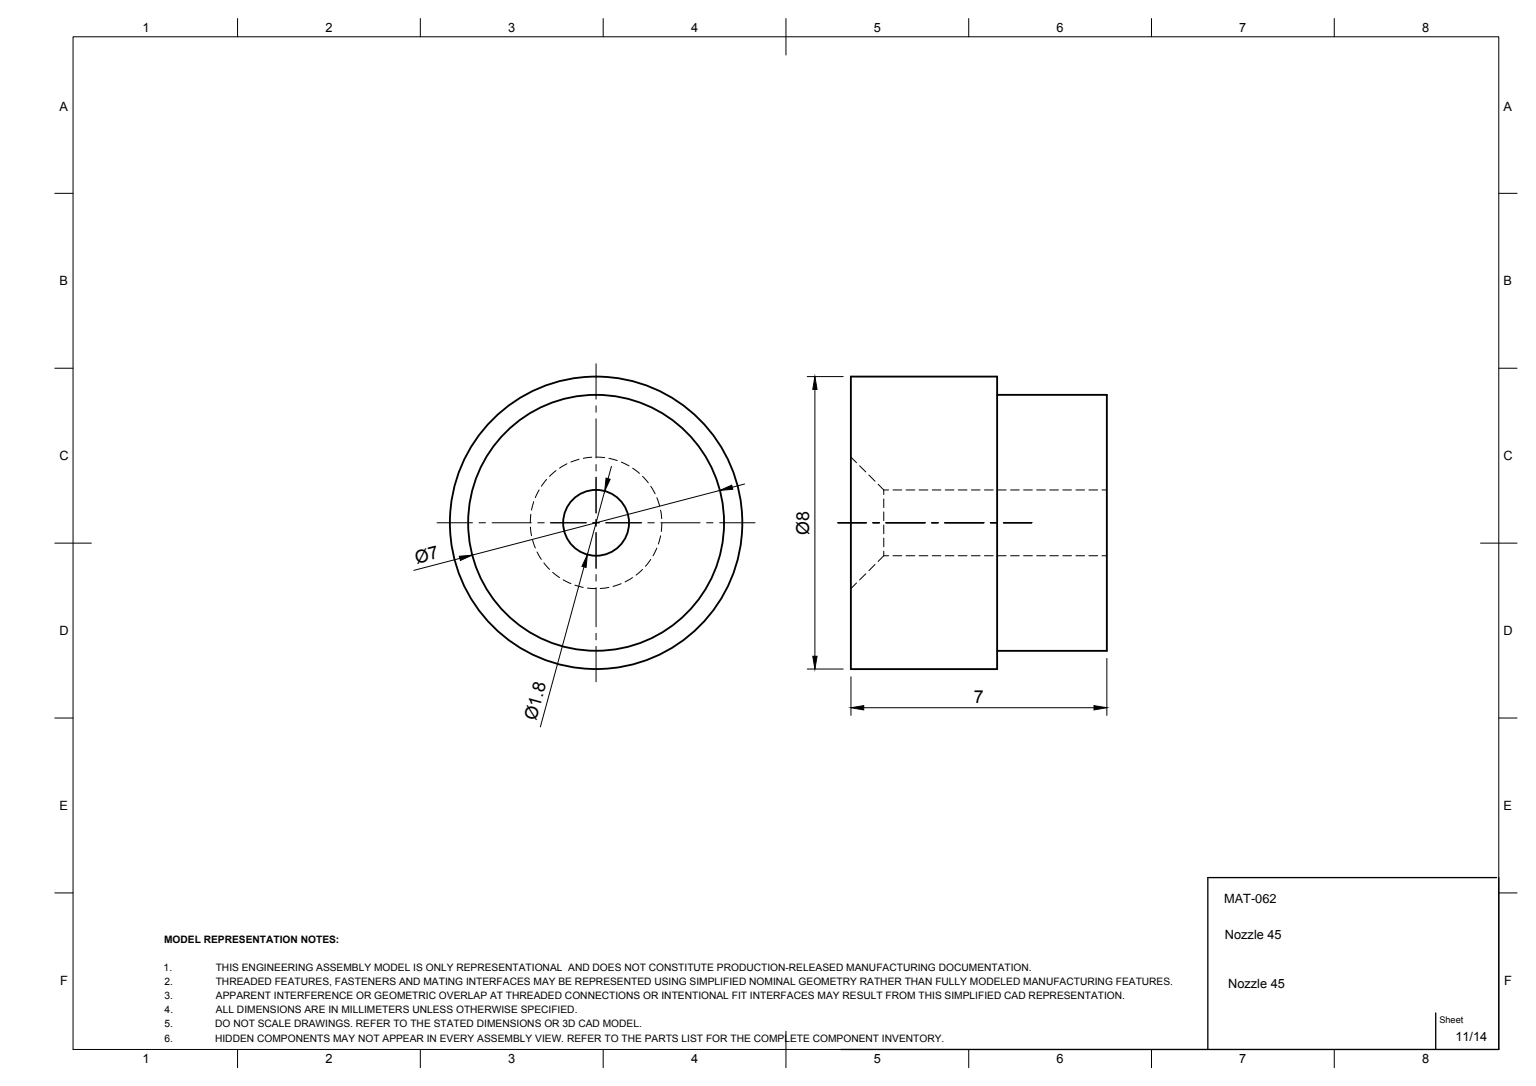
ISO-10303-21;
HEADER;
/* Generated by software containing ST-Developer
 * from STEP Tools, Inc. (www.steptools.com) 
 */

FILE_DESCRIPTION(
/* description */ (''),
/* implementation_level */ '2;1');

FILE_NAME(
/* name */ 'Nozzle 45.step',
/* time_stamp */ '2026-10-24T10:18:25-07:00',
/* author */ (''),
/* organization */ (''),
/* preprocessor_version */ 'ST-DEVELOPER v20.2',
/* originating_system */ 'Autodesk Translation Framework v15.15.0.0',
/* authorisation */ '');

FILE_SCHEMA (('AUTOMOTIVE_DESIGN { 1 0 10303 214 3 1 1 }'));
ENDSEC;

DATA;
#10=MECHANICAL_DESIGN_GEOMETRIC_PRESENTATION_REPRESENTATION('',(#261),#14125);
#195=CONICAL_SURFACE('',#6635,1.8,0.785398163397447);
#232=SHAPE_REPRESENTATION_RELATIONSHIP('SRR','None',#14206,#242);
#242=ADVANCED_BREP_SHAPE_REPRESENTATION('',(#274),#14120);
#261=STYLED_ITEM('',(#14263),#274);
#274=MANIFOLD_SOLID_BREP('Nozzle 45',#6142);
#557=CYLINDRICAL_SURFACE('',#6625,4.00000000000001);
#558=CYLINDRICAL_SURFACE('',#6632,0.899999999999993);
#559=CYLINDRICAL_SURFACE('',#6638,3.50000000000001);
#678=FACE_BOUND('',#1352,.T.);
#679=FACE_BOUND('',#1354,.T.);
#680=FACE_BOUND('',#1358,.T.);
#946=FACE_OUTER_BOUND('',#1350,.T.);
#947=FACE_OUTER_BOUND('',#1351,.T.);
#948=FACE_OUTER_BOUND('',#1353,.T.);
#949=FACE_OUTER_BOUND('',#1355,.T.);
#950=FACE_OUTER_BOUND('',#1356,.T.);
#951=FACE_OUTER_BOUND('',#1357,.T.);
#952=FACE_OUTER_BOUND('',#1359,.T.);
#1350=EDGE_LOOP('',(#5003,#5004,#5005,#5006));
#1351=EDGE_LOOP('',(#5007));
#1352=EDGE_LOOP('',(#5008));
#1353=EDGE_LOOP('',(#5009));
#1354=EDGE_LOOP('',(#5010));
#1355=EDGE_LOOP('',(#5011,#5012,#5013,#5014));
#1356=EDGE_LOOP('',(#5015,#5016,#5017,#5018));
#1357=EDGE_LOOP('',(#5019));
#1358=EDGE_LOOP('',(#5020));
#1359=EDGE_LOOP('',(#5021,#5022,#5023,#5024));
#1706=CIRCLE('',#6626,4.00000000000001);
#1707=CIRCLE('',#6627,4.00000000000001);
#1708=CIRCLE('',#6629,3.50000000000001);
#1709=CIRCLE('',#6631,1.8);
#1710=CIRCLE('',#6633,0.899999999999997);
#1711=CIRCLE('',#6634,0.899999999999995);
#1712=CIRCLE('',#6637,3.50000000000001);
#2042=LINE('',#12244,#2430);
#2043=LINE('',#12256,#2431);
#2044=LINE('',#12259,#2432);
#2045=LINE('',#12264,#2433);
#2430=VECTOR('',#7884,4.00000000000001);
#2431=VECTOR('',#7899,0.899999999999993);
#2432=VECTOR('',#7904,1.8);
#2433=VECTOR('',#7911,3.50000000000002);
#2923=VERTEX_POINT('',#12241);
#2924=VERTEX_POINT('',#12243);
#2925=VERTEX_POINT('',#12247);
#2926=VERTEX_POINT('',#12250);
#2927=VERTEX_POINT('',#12253);
#2928=VERTEX_POINT('',#12255);
#2929=VERTEX_POINT('',#12261);
#3649=EDGE_CURVE('',#2923,#2923,#1706,.T.);
#3650=EDGE_CURVE('',#2923,#2924,#2042,.T.);
#3651=EDGE_CURVE('',#2924,#2924,#1707,.T.);
#3652=EDGE_CURVE('',#2925,#2925,#1708,.T.);
#3653=EDGE_CURVE('',#2926,#2926,#1709,.T.);
#3654=EDGE_CURVE('',#2927,#2927,#1710,.T.);
#3655=EDGE_CURVE('',#2927,#2928,#2043,.T.);
#3656=EDGE_CURVE('',#2928,#2928,#1711,.T.);
#3657=EDGE_CURVE('',#2928,#2926,#2044,.T.);
#3658=EDGE_CURVE('',#2929,#2929,#1712,.T.);
#3659=EDGE_CURVE('',#2925,#2929,#2045,.T.);
#5003=ORIENTED_EDGE('',*,*,#3649,.T.);
#5004=ORIENTED_EDGE('',*,*,#3650,.T.);
#5005=ORIENTED_EDGE('',*,*,#3651,.F.);
#5006=ORIENTED_EDGE('',*,*,#3650,.F.);
#5007=ORIENTED_EDGE('',*,*,#3651,.T.);
#5008=ORIENTED_EDGE('',*,*,#3652,.F.);
#5009=ORIENTED_EDGE('',*,*,#3649,.F.);
#5010=ORIENTED_EDGE('',*,*,#3653,.F.);
#5011=ORIENTED_EDGE('',*,*,#3654,.T.);
#5012=ORIENTED_EDGE('',*,*,#3655,.T.);
#5013=ORIENTED_EDGE('',*,*,#3656,.T.);
#5014=ORIENTED_EDGE('',*,*,#3655,.F.);
#5015=ORIENTED_EDGE('',*,*,#3656,.F.);
#5016=ORIENTED_EDGE('',*,*,#3657,.T.);
#5017=ORIENTED_EDGE('',*,*,#3653,.T.);
#5018=ORIENTED_EDGE('',*,*,#3657,.F.);
#5019=ORIENTED_EDGE('',*,*,#3658,.T.);
#5020=ORIENTED_EDGE('',*,*,#3654,.F.);
#5021=ORIENTED_EDGE('',*,*,#3652,.T.);
#5022=ORIENTED_EDGE('',*,*,#3659,.T.);
#5023=ORIENTED_EDGE('',*,*,#3658,.F.);
#5024=ORIENTED_EDGE('',*,*,#3659,.F.);
#5719=PLANE('',#6628);
#5720=PLANE('',#6630);
#5721=PLANE('',#6636);
#5995=ADVANCED_FACE('',(#946),#557,.T.);
#5996=ADVANCED_FACE('',(#947,#678),#5719,.T.);
#5997=ADVANCED_FACE('',(#948,#679),#5720,.F.);
#5998=ADVANCED_FACE('',(#949),#558,.F.);
#5999=ADVANCED_FACE('',(#950),#195,.F.);
#6000=ADVANCED_FACE('',(#951,#680),#5721,.T.);
#6001=ADVANCED_FACE('',(#952),#559,.T.);
#6142=CLOSED_SHELL('',(#5995,#5996,#5997,#5998,#5999,#6000,#6001));
#6624=AXIS2_PLACEMENT_3D('',#12239,#7878,#7879);
#6625=AXIS2_PLACEMENT_3D('',#12240,#7880,#7881);
#6626=AXIS2_PLACEMENT_3D('',#12242,#7882,#7883);
#6627=AXIS2_PLACEMENT_3D('',#12245,#7885,#7886);
#6628=AXIS2_PLACEMENT_3D('',#12246,#7887,#7888);
#6629=AXIS2_PLACEMENT_3D('',#12248,#7889,#7890);
#6630=AXIS2_PLACEMENT_3D('',#12249,#7891,#7892);
#6631=AXIS2_PLACEMENT_3D('',#12251,#7893,#7894);
#6632=AXIS2_PLACEMENT_3D('',#12252,#7895,#7896);
#6633=AXIS2_PLACEMENT_3D('',#12254,#7897,#7898);
#6634=AXIS2_PLACEMENT_3D('',#12257,#7900,#7901);
#6635=AXIS2_PLACEMENT_3D('',#12258,#7902,#7903);
#6636=AXIS2_PLACEMENT_3D('',#12260,#7905,#7906);
#6637=AXIS2_PLACEMENT_3D('',#12262,#7907,#7908);
#6638=AXIS2_PLACEMENT_3D('',#12263,#7909,#7910);
#7878=DIRECTION('axis',(0.,0.,1.));
#7879=DIRECTION('refdir',(1.,0.,0.));
#7880=DIRECTION('center_axis',(-0.612372435695796,0.707106781186546,-0.353553390593275));
#7881=DIRECTION('ref_axis',(-0.755928946018453,-0.654653670707979,0.));
#7882=DIRECTION('center_axis',(0.612372435695796,-0.707106781186546,0.353553390593275));
#7883=DIRECTION('ref_axis',(0.755928946018453,0.654653670707979,0.));
#7884=DIRECTION('',(0.612372435695796,-0.707106781186546,0.353553390593275));
#7885=DIRECTION('center_axis',(0.612372435695796,-0.707106781186546,0.353553390593275));
#7886=DIRECTION('ref_axis',(0.755928946018453,0.654653670707979,0.));
#7887=DIRECTION('center_axis',(0.612372435695796,-0.707106781186546,0.353553390593275));
#7888=DIRECTION('ref_axis',(0.5,0.,-0.866025403784438));
#7889=DIRECTION('center_axis',(0.612372435695796,-0.707106781186546,0.353553390593275));
#7890=DIRECTION('ref_axis',(0.755928946018453,0.654653670707979,0.));
#7891=DIRECTION('center_axis',(0.612372435695796,-0.707106781186546,0.353553390593275));
#7892=DIRECTION('ref_axis',(0.5,0.,-0.866025403784438));
#7893=DIRECTION('center_axis',(-0.612372435695796,0.707106781186546,-0.353553390593275));
#7894=DIRECTION('ref_axis',(-0.755928946018453,-0.654653670707979,0.));
#7895=DIRECTION('center_axis',(-0.612372435695796,0.707106781186546,-0.353553390593275));
#7896=DIRECTION('ref_axis',(-0.755928946018453,-0.654653670707979,0.));
#7897=DIRECTION('center_axis',(0.612372435695796,-0.707106781186546,0.353553390593275));
#7898=DIRECTION('ref_axis',(0.755928946018453,0.654653670707979,0.));
#7899=DIRECTION('',(-0.612372435695796,0.707106781186546,-0.353553390593275));
#7900=DIRECTION('center_axis',(-0.612372435695796,0.707106781186546,-0.353553390593275));
#7901=DIRECTION('ref_axis',(-0.755928946018453,-0.654653670707979,0.));
#7902=DIRECTION('center_axis',(-0.612372435695796,0.707106781186546,-0.353553390593275));
#7903=DIRECTION('ref_axis',(-0.755928946018453,-0.654653670707979,0.));
#7904=DIRECTION('',(0.101509781932626,0.962910049886276,-0.250000000000001));
#7905=DIRECTION('center_axis',(0.612372435695796,-0.707106781186546,0.353553390593275));
#7906=DIRECTION('ref_axis',(0.5,0.,-0.866025403784438));
#7907=DIRECTION('center_axis',(0.612372435695796,-0.707106781186546,0.353553390593275));
#7908=DIRECTION('ref_axis',(0.755928946018453,0.654653670707979,0.));
#7909=DIRECTION('center_axis',(-0.612372435695796,0.707106781186546,-0.353553390593275));
#7910=DIRECTION('ref_axis',(-0.755928946018453,-0.654653670707979,0.));
#7911=DIRECTION('',(0.612372435695796,-0.707106781186546,0.353553390593275));
#12239=CARTESIAN_POINT('',(0.,0.,0.));
#12240=CARTESIAN_POINT('Origin',(-116.12807069331,130.343145750508,-79.0465728752519));
#12241=CARTESIAN_POINT('',(-115.553844652019,135.790187558086,-80.460786437625));
#12242=CARTESIAN_POINT('Origin',(-118.577560436093,133.171572875254,-80.460786437625));
#12243=CARTESIAN_POINT('',(-113.104354909236,132.96176043334,-79.0465728752519));
#12244=CARTESIAN_POINT('',(-113.104354909236,132.96176043334,-79.0465728752519));
#12245=CARTESIAN_POINT('Origin',(-116.12807069331,130.343145750508,-79.0465728752519));
#12246=CARTESIAN_POINT('Origin',(-116.12807069331,130.343145750508,-79.0465728752519));
#12247=CARTESIAN_POINT('',(-113.482319382245,132.634433597986,-79.0465728752519));
#12248=CARTESIAN_POINT('Origin',(-116.12807069331,130.343145750508,-79.0465728752519));
#12249=CARTESIAN_POINT('Origin',(-118.577560436093,133.171572875254,-80.460786437625));
#12250=CARTESIAN_POINT('',(-117.21688833326,134.349949482528,-80.460786437625));
#12251=CARTESIAN_POINT('Origin',(-118.577560436093,133.171572875254,-80.460786437625));
#12252=CARTESIAN_POINT('Origin',(-118.577560436093,133.171572875254,-80.460786437625));
#12253=CARTESIAN_POINT('',(-113.610617334806,128.811013710585,-77.9859127034721));
#12254=CARTESIAN_POINT('Origin',(-114.290953386223,128.221825406948,-77.9859127034721));
#12255=CARTESIAN_POINT('',(-117.34608919255,133.124365075823,-80.1425883860911));
#12256=CARTESIAN_POINT('',(-117.897224384677,133.760761178891,-80.460786437625));
#12257=CARTESIAN_POINT('Origin',(-118.026425243967,132.535176772186,-80.1425883860911));
#12258=CARTESIAN_POINT('Origin',(-118.577560436093,133.171572875254,-80.460786437625));
#12259=CARTESIAN_POINT('',(-117.21688833326,134.349949482528,-80.460786437625));
#12260=CARTESIAN_POINT('Origin',(-114.290953386223,128.221825406948,-77.9859127034721));
#12261=CARTESIAN_POINT('',(-111.645202075158,130.513113254426,-77.9859127034721));
#12262=CARTESIAN_POINT('Origin',(-114.290953386223,128.221825406948,-77.9859127034721));
#12263=CARTESIAN_POINT('Origin',(-114.290953386223,128.221825406948,-77.9859127034721));
#12264=CARTESIAN_POINT('',(-111.645202075158,130.513113254426,-77.9859127034721));
#14107=UNCERTAINTY_MEASURE_WITH_UNIT(LENGTH_MEASURE(0.01),#14126,
'DISTANCE_ACCURACY_VALUE',
'Maximum model space distance between geometric entities at asserted c
onnectivities');
#14112=UNCERTAINTY_MEASURE_WITH_UNIT(LENGTH_MEASURE(0.01),#14126,
'DISTANCE_ACCURACY_VALUE',
'Maximum model space distance between geometric entities at asserted c
onnectivities');
#14120=(
GEOMETRIC_REPRESENTATION_CONTEXT(3)
GLOBAL_UNCERTAINTY_ASSIGNED_CONTEXT((#14107))
GLOBAL_UNIT_ASSIGNED_CONTEXT((#14126,#14128,#14129))
REPRESENTATION_CONTEXT('','3D')
);
#14125=(
GEOMETRIC_REPRESENTATION_CONTEXT(3)
GLOBAL_UNCERTAINTY_ASSIGNED_CONTEXT((#14112))
GLOBAL_UNIT_ASSIGNED_CONTEXT((#14126,#14128,#14129))
REPRESENTATION_CONTEXT('','3D')
);
#14126=(
LENGTH_UNIT()
NAMED_UNIT(*)
SI_UNIT(.MILLI.,.METRE.)
);
#14128=(
NAMED_UNIT(*)
PLANE_ANGLE_UNIT()
SI_UNIT($,.RADIAN.)
);
#14129=(
NAMED_UNIT(*)
SI_UNIT($,.STERADIAN.)
SOLID_ANGLE_UNIT()
);
#14137=SHAPE_DEFINITION_REPRESENTATION(#14149,#14206);
#14149=PRODUCT_DEFINITION_SHAPE('',$,#14219);
#14206=SHAPE_REPRESENTATION('',(#6624),#14120);
#14211=PRODUCT_DEFINITION_CONTEXT('part definition',#14249,'design');
#14219=PRODUCT_DEFINITION('Nozzle 45','Nozzle 45',#14231,#14211);
#14231=PRODUCT_DEFINITION_FORMATION('',$,#14258);
#14249=APPLICATION_CONTEXT(
'Core Data for Automotive Mechanical Design Process');
#14250=PRODUCT_CONTEXT('part definition',#14249,'mechanical');
#14258=PRODUCT('Nozzle 45','Nozzle 45',$,(#14250));
#14263=PRESENTATION_STYLE_ASSIGNMENT((#14265));
#14265=SURFACE_STYLE_USAGE(.BOTH.,#14267);
#14267=SURFACE_SIDE_STYLE('',(#14269));
#14269=SURFACE_STYLE_FILL_AREA(#14271);
#14271=FILL_AREA_STYLE('Steel - Satin',(#14273));
#14273=FILL_AREA_STYLE_COLOUR('Steel - Satin',#14275);
#14275=COLOUR_RGB('Steel - Satin',0.627450980392157,0.627450980392157,0.627450980392157);
ENDSEC;
END-ISO-10303-21;
